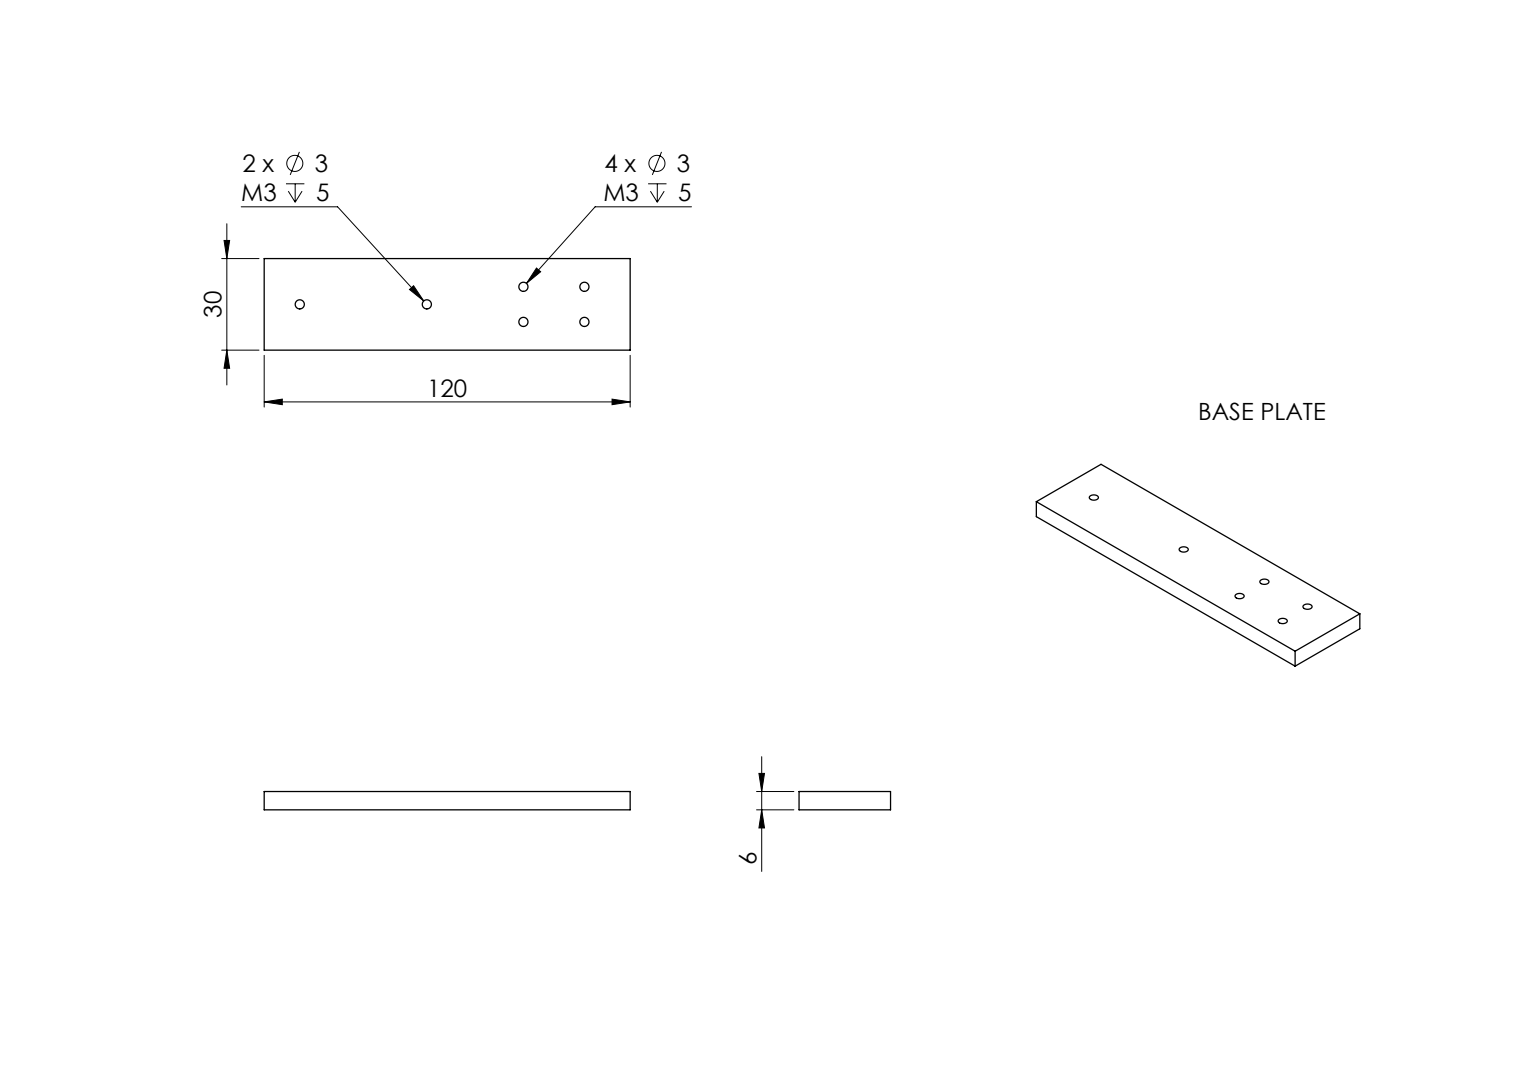
ISO-10303-21;
HEADER;
FILE_DESCRIPTION (('STEP AP214'),
    '1' );
FILE_NAME ('base plate.step',
    '2026-10-26T05:17:54',
    ( '' ),
    ( '' ),
    'SwSTEP 2.0',
    'SolidWorks 2026',
    '' );
FILE_SCHEMA (( 'AUTOMOTIVE_DESIGN' ));
ENDSEC;

DATA;
#8=DIRECTION ( 'NONE',  ( -0.000000000000000000, 1.000000000000000000, -0.000000000000000000 ) ) ;
#20=SURFACE_STYLE_FILL_AREA ( #10773 ) ;
#32=CARTESIAN_POINT ( 'NONE',  ( 45.00000000000000000, 0.000000000000000000, -4.249999999999998224 ) ) ;
#39=VERTEX_POINT ( 'NONE', #7644 ) ;
#40=COLOUR_RGB ( '',0.8941176470588234615, 0.8941176470588234615, 0.8941176470588234615 ) ;
#57=EDGE_CURVE ( 'NONE', #11292, #8351, #9858, .T. ) ;
#75=FACE_BOUND ( 'NONE', #11702, .T. ) ;
#138=DIRECTION ( 'NONE',  ( 0.000000000000000000, 0.000000000000000000, 1.000000000000000000 ) ) ;
#139=DIRECTION ( 'NONE',  ( 0.000000000000000000, -0.000000000000000000, -1.000000000000000000 ) ) ;
#141=ADVANCED_FACE ( 'NONE', ( #3852 ), #10839, .F. ) ;
#168=EDGE_CURVE ( 'NONE', #9993, #9602, #10963, .T. ) ;
#174=EDGE_LOOP ( 'NONE', ( #6858, #8002, #3578, #927 ) ) ;
#212=CARTESIAN_POINT ( 'NONE',  ( -48.33333333333332860, -5.000000000000000000, -1.500000000000003109 ) ) ;
#223=ADVANCED_FACE ( 'NONE', ( #9797 ), #3264, .F. ) ;
#226=DIRECTION ( 'NONE',  ( -0.000000000000000000, 1.000000000000000000, -0.000000000000000000 ) ) ;
#230=ORIENTED_EDGE ( 'NONE', *, *, #426, .T. ) ;
#248=DIRECTION ( 'NONE',  ( 1.049727191973305517E-16, 0.5150380737757253025, -0.8571673013836857979 ) ) ;
#266=LINE ( 'NONE', #12261, #1845 ) ;
#305=ORIENTED_EDGE ( 'NONE', *, *, #8048, .F. ) ;
#309=VERTEX_POINT ( 'NONE', #6189 ) ;
#369=AXIS2_PLACEMENT_3D ( 'NONE', #12355, #9278, #12488 ) ;
#376=VERTEX_POINT ( 'NONE', #8487 ) ;
#382=CARTESIAN_POINT ( 'NONE',  ( 60.00000000000000000, -6.000000000000000000, 15.00000000000000000 ) ) ;
#426=EDGE_CURVE ( 'NONE', #11653, #6806, #2729, .T. ) ;
#432=DIRECTION ( 'NONE',  ( 0.000000000000000000, 0.000000000000000000, 1.000000000000000000 ) ) ;
#469=DIRECTION ( 'NONE',  ( -0.000000000000000000, 1.000000000000000000, -0.000000000000000000 ) ) ;
#487=DIRECTION ( 'NONE',  ( -0.000000000000000000, 1.000000000000000000, -0.000000000000000000 ) ) ;
#502=AXIS2_PLACEMENT_3D ( 'NONE', #7934, #12717, #11921 ) ;
#511=CARTESIAN_POINT ( 'NONE',  ( -6.666666666666660745, 0.000000000000000000, 0.000000000000000000 ) ) ;
#549=VECTOR ( 'NONE', #1621, 1000.000000000000000 ) ;
#554=DIRECTION ( 'NONE',  ( 0.000000000000000000, 0.000000000000000000, 1.000000000000000000 ) ) ;
#561=VECTOR ( 'NONE', #4344, 999.9999999999998863 ) ;
#572=DIRECTION ( 'NONE',  ( -1.000000000000000000, 0.000000000000000000, 0.000000000000000000 ) ) ;
#603=DIRECTION ( 'NONE',  ( 0.000000000000000000, 0.5150380737757253025, 0.8571673013836857979 ) ) ;
#642=ORIENTED_EDGE ( 'NONE', *, *, #5141, .F. ) ;
#646=DIRECTION ( 'NONE',  ( 0.000000000000000000, 0.000000000000000000, 1.000000000000000000 ) ) ;
#661=AXIS2_PLACEMENT_3D ( 'NONE', #10121, #1470, #8480 ) ;
#670=PLANE ( 'NONE',  #6171 ) ;
#691=CARTESIAN_POINT ( 'NONE',  ( 25.00000000000000355, 0.000000000000000000, 4.249999999999998224 ) ) ;
#711=DIRECTION ( 'NONE',  ( 0.000000000000000000, 0.5150380737757253025, 0.8571673013836857979 ) ) ;
#714=AXIS2_PLACEMENT_3D ( 'NONE', #11287, #12341, #11156 ) ;
#718=VERTEX_POINT ( 'NONE', #4225 ) ;
#732=CIRCLE ( 'NONE', #5327, 1.499999999999999556 ) ;
#743=CIRCLE ( 'NONE', #2637, 1.500000000000001332 ) ;
#761=( LENGTH_UNIT ( ) NAMED_UNIT ( * ) SI_UNIT ( .MILLI., .METRE. ) );
#827=CIRCLE ( 'NONE', #4601, 1.500000000000001332 ) ;
#829=ORIENTED_EDGE ( 'NONE', *, *, #3040, .F. ) ;
#834=EDGE_LOOP ( 'NONE', ( #3807, #9213, #11904 ) ) ;
#835=VERTEX_POINT ( 'NONE', #7421 ) ;
#836=CYLINDRICAL_SURFACE ( 'NONE', #9008, 1.500000000000001332 ) ;
#842=ORIENTED_EDGE ( 'NONE', *, *, #4723, .T. ) ;
#873=ADVANCED_FACE ( 'NONE', ( #1662 ), #6562, .F. ) ;
#880=CARTESIAN_POINT ( 'NONE',  ( 60.00000000000000000, 0.000000000000000000, 15.00000000000000000 ) ) ;
#882=( NAMED_UNIT ( * ) SI_UNIT ( $, .STERADIAN. ) SOLID_ANGLE_UNIT ( ) );
#886=CARTESIAN_POINT ( 'NONE',  ( -60.00000000000000000, -6.000000000000000000, 14.99999999999999645 ) ) ;
#921=AXIS2_PLACEMENT_3D ( 'NONE', #2490, #6466, #10462 ) ;
#927=ORIENTED_EDGE ( 'NONE', *, *, #11531, .F. ) ;
#947=SURFACE_SIDE_STYLE ('',( #20 ) ) ;
#961=DIRECTION ( 'NONE',  ( -0.000000000000000000, 1.000000000000000000, -0.000000000000000000 ) ) ;
#964=CARTESIAN_POINT ( 'NONE',  ( 25.00000000000000355, 0.000000000000000000, 5.750000000000000000 ) ) ;
#965=ORIENTED_EDGE ( 'NONE', *, *, #11531, .T. ) ;
#968=ORIENTED_EDGE ( 'NONE', *, *, #12311, .F. ) ;
#991=AXIS2_PLACEMENT_3D ( 'NONE', #6237, #12192, #2261 ) ;
#992=VERTEX_POINT ( 'NONE', #5842 ) ;
#1021=ORIENTED_EDGE ( 'NONE', *, *, #1157, .F. ) ;
#1080=CARTESIAN_POINT ( 'NONE',  ( 45.00000000000000000, -5.000000000000000000, -5.750000000000000000 ) ) ;
#1123=VECTOR ( 'NONE', #2979, 1000.000000000000000 ) ;
#1131=CIRCLE ( 'NONE', #10551, 1.500000000000001332 ) ;
#1145=CARTESIAN_POINT ( 'NONE',  ( 25.00000000000000355, -5.901290925839664858, 5.750000000000000000 ) ) ;
#1149=AXIS2_PLACEMENT_3D ( 'NONE', #11024, #8159, #2079 ) ;
#1150=ORIENTED_EDGE ( 'NONE', *, *, #3390, .T. ) ;
#1157=EDGE_CURVE ( 'NONE', #11476, #11262, #3029, .T. ) ;
#1162=AXIS2_PLACEMENT_3D ( 'NONE', #1080, #9331, #5271 ) ;
#1190=ORIENTED_EDGE ( 'NONE', *, *, #12704, .T. ) ;
#1200=EDGE_CURVE ( 'NONE', #11292, #11250, #10783, .T. ) ;
#1210=VECTOR ( 'NONE', #2174, 1000.000000000000000 ) ;
#1212=ORIENTED_EDGE ( 'NONE', *, *, #4918, .T. ) ;
#1215=FACE_OUTER_BOUND ( 'NONE', #9863, .T. ) ;
#1219=ORIENTED_EDGE ( 'NONE', *, *, #11969, .T. ) ;
#1227=AXIS2_PLACEMENT_3D ( 'NONE', #3244, #11210, #139 ) ;
#1234=ORIENTED_EDGE ( 'NONE', *, *, #11061, .F. ) ;
#1244=ORIENTED_EDGE ( 'NONE', *, *, #5393, .F. ) ;
#1248=AXIS2_PLACEMENT_3D ( 'NONE', #1741, #5729, #4754 ) ;
#1272=EDGE_CURVE ( 'NONE', #9602, #3240, #4770, .T. ) ;
#1314=LINE ( 'NONE', #10350, #3761 ) ;
#1322=ADVANCED_FACE ( 'NONE', ( #5552 ), #9549, .T. ) ;
#1356=DIRECTION ( 'NONE',  ( -0.000000000000000000, 1.000000000000000000, -0.000000000000000000 ) ) ;
#1379=AXIS2_PLACEMENT_3D ( 'NONE', #8945, #961, #3988 ) ;
#1413=VERTEX_POINT ( 'NONE', #1886 ) ;
#1426=VECTOR ( 'NONE', #3530, 999.9999999999998863 ) ;
#1427=VERTEX_POINT ( 'NONE', #4956 ) ;
#1429=ORIENTED_EDGE ( 'NONE', *, *, #5239, .T. ) ;
#1450=DIRECTION ( 'NONE',  ( -0.000000000000000000, 1.000000000000000000, -0.000000000000000000 ) ) ;
#1453=VECTOR ( 'NONE', #6804, 1000.000000000000000 ) ;
#1458=ADVANCED_FACE ( 'NONE', ( #4045 ), #9800, .F. ) ;
#1461=CIRCLE ( 'NONE', #10650, 1.499999999999999556 ) ;
#1463=DIRECTION ( 'NONE',  ( -0.000000000000000000, 1.000000000000000000, -0.000000000000000000 ) ) ;
#1465=FACE_OUTER_BOUND ( 'NONE', #4679, .T. ) ;
#1470=DIRECTION ( 'NONE',  ( -0.000000000000000000, 1.000000000000000000, -0.000000000000000000 ) ) ;
#1475=DIRECTION ( 'NONE',  ( -0.000000000000000000, 1.000000000000000000, -0.000000000000000000 ) ) ;
#1500=CIRCLE ( 'NONE', #661, 1.500000000000001332 ) ;
#1512=ORIENTED_EDGE ( 'NONE', *, *, #4521, .T. ) ;
#1514=EDGE_LOOP ( 'NONE', ( #2019, #3145, #9148, #1219 ) ) ;
#1544=EDGE_CURVE ( 'NONE', #3240, #4006, #11813, .T. ) ;
#1580=AXIS2_PLACEMENT_3D ( 'NONE', #10565, #12391, #2459 ) ;
#1611=CARTESIAN_POINT ( 'NONE',  ( -48.33333333333332860, 0.000000000000000000, 1.499999999999999556 ) ) ;
#1621=DIRECTION ( 'NONE',  ( 1.049727191973305763E-16, 0.5150380737757249694, -0.8571673013836860200 ) ) ;
#1628=CIRCLE ( 'NONE', #6230, 1.500000000000001332 ) ;
#1639=CIRCLE ( 'NONE', #4977, 1.499999999999999556 ) ;
#1660=DIRECTION ( 'NONE',  ( -0.000000000000000000, 1.000000000000000000, -0.000000000000000000 ) ) ;
#1662=FACE_OUTER_BOUND ( 'NONE', #1514, .T. ) ;
#1692=VERTEX_POINT ( 'NONE', #8490 ) ;
#1702=VECTOR ( 'NONE', #1846, 1000.000000000000000 ) ;
#1729=EDGE_CURVE ( 'NONE', #3927, #7180, #732, .T. ) ;
#1741=CARTESIAN_POINT ( 'NONE',  ( 45.00000000000000000, 0.000000000000000000, 5.750000000000000888 ) ) ;
#1762=PRODUCT_DEFINITION_FORMATION_WITH_SPECIFIED_SOURCE ( 'ANY', '', #11480, .NOT_KNOWN. ) ;
#1813=EDGE_CURVE ( 'NONE', #835, #10173, #10698, .T. ) ;
#1836=CARTESIAN_POINT ( 'NONE',  ( 25.00000000000000355, -5.000000000000000000, 4.249999999999998224 ) ) ;
#1837=EDGE_LOOP ( 'NONE', ( #829, #11058 ) ) ;
#1845=VECTOR ( 'NONE', #3309, 999.9999999999998863 ) ;
#1846=DIRECTION ( 'NONE',  ( -0.000000000000000000, 1.000000000000000000, -0.000000000000000000 ) ) ;
#1850=ADVANCED_FACE ( 'NONE', ( #8989 ), #5792, .F. ) ;
#1861=EDGE_CURVE ( 'NONE', #6806, #1692, #2861, .T. ) ;
#1886=CARTESIAN_POINT ( 'NONE',  ( 45.00000000000000000, -5.000000000000000000, -4.249999999999998224 ) ) ;
#1894=VERTEX_POINT ( 'NONE', #8017 ) ;
#1904=AXIS2_PLACEMENT_3D ( 'NONE', #12320, #3368, #6359 ) ;
#1943=ADVANCED_FACE ( 'NONE', ( #7953 ), #12793, .F. ) ;
#1957=EDGE_LOOP ( 'NONE', ( #2157, #3202 ) ) ;
#1966=CARTESIAN_POINT ( 'NONE',  ( 60.00000000000000000, -6.000000000000000000, 15.00000000000000000 ) ) ;
#1967=ORIENTED_EDGE ( 'NONE', *, *, #5239, .F. ) ;
#1990=LINE ( 'NONE', #9109, #3375 ) ;
#2019=ORIENTED_EDGE ( 'NONE', *, *, #7283, .F. ) ;
#2050=CIRCLE ( 'NONE', #4767, 1.500000000000001332 ) ;
#2073=( LENGTH_UNIT ( ) NAMED_UNIT ( * ) SI_UNIT ( .MILLI., .METRE. ) );
#2079=DIRECTION ( 'NONE',  ( 0.000000000000000000, 0.000000000000000000, 1.000000000000000000 ) ) ;
#2096=VERTEX_POINT ( 'NONE', #3116 ) ;
#2102=LINE ( 'NONE', #12040, #7594 ) ;
#2111=ORIENTED_EDGE ( 'NONE', *, *, #9460, .T. ) ;
#2112=VECTOR ( 'NONE', #11928, 1000.000000000000000 ) ;
#2127=EDGE_CURVE ( 'NONE', #718, #309, #8213, .T. ) ;
#2142=DIRECTION ( 'NONE',  ( 0.000000000000000000, 0.000000000000000000, 1.000000000000000000 ) ) ;
#2143=EDGE_CURVE ( 'NONE', #10857, #8362, #12026, .T. ) ;
#2157=ORIENTED_EDGE ( 'NONE', *, *, #5870, .F. ) ;
#2167=ORIENTED_EDGE ( 'NONE', *, *, #4353, .T. ) ;
#2174=DIRECTION ( 'NONE',  ( 0.000000000000000000, 0.000000000000000000, -1.000000000000000000 ) ) ;
#2201=ADVANCED_FACE ( 'NONE', ( #1465 ), #670, .T. ) ;
#2249=ORIENTED_EDGE ( 'NONE', *, *, #57, .T. ) ;
#2250=EDGE_CURVE ( 'NONE', #2096, #9602, #2849, .T. ) ;
#2261=DIRECTION ( 'NONE',  ( 0.000000000000000000, 0.000000000000000000, 1.000000000000000000 ) ) ;
#2262=PLANE ( 'NONE',  #1227 ) ;
#2292=PLANE ( 'NONE',  #369 ) ;
#2299=EDGE_CURVE ( 'NONE', #4333, #3861, #12859, .T. ) ;
#2307=LINE ( 'NONE', #8254, #11740 ) ;
#2326=CARTESIAN_POINT ( 'NONE',  ( 25.00000000000000355, 0.000000000000000000, 7.250000000000000888 ) ) ;
#2376=ORIENTED_EDGE ( 'NONE', *, *, #5336, .F. ) ;
#2431=DIRECTION ( 'NONE',  ( 0.000000000000000000, 0.000000000000000000, 1.000000000000000000 ) ) ;
#2451=DIRECTION ( 'NONE',  ( -0.000000000000000000, 1.000000000000000000, -0.000000000000000000 ) ) ;
#2459=DIRECTION ( 'NONE',  ( 0.000000000000000000, 0.000000000000000000, 1.000000000000000000 ) ) ;
#2463=DIRECTION ( 'NONE',  ( -0.000000000000000000, 1.000000000000000000, -0.000000000000000000 ) ) ;
#2470=CARTESIAN_POINT ( 'NONE',  ( 25.00000000000000355, -5.000000000000000000, -4.249999999999998224 ) ) ;
#2480=ORIENTED_EDGE ( 'NONE', *, *, #8048, .T. ) ;
#2490=CARTESIAN_POINT ( 'NONE',  ( 45.00000000000000000, 0.000000000000000000, -5.750000000000000000 ) ) ;
#2515=APPLICATION_CONTEXT ( 'automotive_design' ) ;
#2522=CARTESIAN_POINT ( 'NONE',  ( -48.33333333333332860, 0.000000000000000000, -1.734723475976807094E-15 ) ) ;
#2523=DIRECTION ( 'NONE',  ( 0.000000000000000000, -0.000000000000000000, -1.000000000000000000 ) ) ;
#2528=AXIS2_PLACEMENT_3D ( 'NONE', #6434, #12203, #4480 ) ;
#2585=DIRECTION ( 'NONE',  ( -0.000000000000000000, 1.000000000000000000, -0.000000000000000000 ) ) ;
#2600=FACE_OUTER_BOUND ( 'NONE', #10043, .T. ) ;
#2636=EDGE_CURVE ( 'NONE', #6649, #7180, #12447, .T. ) ;
#2637=AXIS2_PLACEMENT_3D ( 'NONE', #9130, #12147, #10308 ) ;
#2658=ORIENTED_EDGE ( 'NONE', *, *, #1813, .T. ) ;
#2697=EDGE_CURVE ( 'NONE', #8362, #12765, #2102, .T. ) ;
#2729=LINE ( 'NONE', #2470, #11141 ) ;
#2730=DIRECTION ( 'NONE',  ( -1.000000000000000000, -0.000000000000000000, -0.000000000000000000 ) ) ;
#2740=FACE_OUTER_BOUND ( 'NONE', #11021, .T. ) ;
#2763=APPLICATION_CONTEXT ( 'automotive_design' ) ;
#2809=ORIENTED_EDGE ( 'NONE', *, *, #5336, .T. ) ;
#2825=ORIENTED_EDGE ( 'NONE', *, *, #3804, .F. ) ;
#2849=CIRCLE ( 'NONE', #10145, 1.500000000000001332 ) ;
#2861=LINE ( 'NONE', #5855, #8272 ) ;
#2868=CIRCLE ( 'NONE', #6403, 1.500000000000001332 ) ;
#2884=EDGE_LOOP ( 'NONE', ( #11242, #3591, #10722 ) ) ;
#2902=FACE_OUTER_BOUND ( 'NONE', #7339, .T. ) ;
#2922=DIRECTION ( 'NONE',  ( -0.000000000000000000, 1.000000000000000000, -0.000000000000000000 ) ) ;
#2941=LINE ( 'NONE', #32, #8499 ) ;
#2956=ORIENTED_EDGE ( 'NONE', *, *, #9180, .F. ) ;
#2970=VERTEX_POINT ( 'NONE', #1145 ) ;
#2979=DIRECTION ( 'NONE',  ( -0.000000000000000000, -0.000000000000000000, 1.000000000000000000 ) ) ;
#3018=CARTESIAN_POINT ( 'NONE',  ( 45.00000000000000000, 0.000000000000000000, -7.250000000000000888 ) ) ;
#3021=CIRCLE ( 'NONE', #5091, 1.500000000000001332 ) ;
#3029=CIRCLE ( 'NONE', #921, 1.500000000000001332 ) ;
#3040=EDGE_CURVE ( 'NONE', #4006, #3240, #743, .T. ) ;
#3041=ADVANCED_FACE ( 'NONE', ( #1215 ), #8221, .F. ) ;
#3048=EDGE_CURVE ( 'NONE', #1413, #39, #9521, .T. ) ;
#3063=CARTESIAN_POINT ( 'NONE',  ( 25.00000000000000355, 0.000000000000000000, -5.750000000000000000 ) ) ;
#3088=ORIENTED_EDGE ( 'NONE', *, *, #9280, .F. ) ;
#3110=DIRECTION ( 'NONE',  ( -0.000000000000000000, 1.000000000000000000, -0.000000000000000000 ) ) ;
#3113=CIRCLE ( 'NONE', #3943, 1.500000000000001332 ) ;
#3116=CARTESIAN_POINT ( 'NONE',  ( 45.00000000000000000, -5.000000000000000000, 7.250000000000001776 ) ) ;
#3117=AXIS2_PLACEMENT_3D ( 'NONE', #3412, #3288, #2431 ) ;
#3140=EDGE_LOOP ( 'NONE', ( #3540, #7051, #10160 ) ) ;
#3145=ORIENTED_EDGE ( 'NONE', *, *, #2299, .F. ) ;
#3171=ORIENTED_EDGE ( 'NONE', *, *, #4593, .F. ) ;
#3199=ORIENTED_EDGE ( 'NONE', *, *, #1813, .F. ) ;
#3202=ORIENTED_EDGE ( 'NONE', *, *, #10109, .F. ) ;
#3229=ORIENTED_EDGE ( 'NONE', *, *, #4593, .T. ) ;
#3240=VERTEX_POINT ( 'NONE', #7653 ) ;
#3244=CARTESIAN_POINT ( 'NONE',  ( 0.000000000000000000, 0.000000000000000000, 0.000000000000000000 ) ) ;
#3250=DIRECTION ( 'NONE',  ( 0.000000000000000000, 0.5150380737757255245, 0.8571673013836856869 ) ) ;
#3263=AXIS2_PLACEMENT_3D ( 'NONE', #4676, #7551, #8541 ) ;
#3264=CYLINDRICAL_SURFACE ( 'NONE', #9272, 1.500000000000001332 ) ;
#3288=DIRECTION ( 'NONE',  ( -0.000000000000000000, 1.000000000000000000, -0.000000000000000000 ) ) ;
#3289=ORIENTED_EDGE ( 'NONE', *, *, #8865, .F. ) ;
#3309=DIRECTION ( 'NONE',  ( 1.049727191973305517E-16, 0.5150380737757253025, -0.8571673013836857979 ) ) ;
#3310=FACE_BOUND ( 'NONE', #1957, .T. ) ;
#3316=FACE_OUTER_BOUND ( 'NONE', #7620, .T. ) ;
#3322=ORIENTED_EDGE ( 'NONE', *, *, #2636, .F. ) ;
#3328=EDGE_CURVE ( 'NONE', #1894, #4333, #10846, .T. ) ;
#3362=ADVANCED_FACE ( 'NONE', ( #9995 ), #9730, .F. ) ;
#3368=DIRECTION ( 'NONE',  ( -0.000000000000000000, 1.000000000000000000, -0.000000000000000000 ) ) ;
#3375=VECTOR ( 'NONE', #4085, 1000.000000000000000 ) ;
#3383=EDGE_LOOP ( 'NONE', ( #1967, #230, #5298 ) ) ;
#3390=EDGE_CURVE ( 'NONE', #1413, #11262, #2941, .T. ) ;
#3412=CARTESIAN_POINT ( 'NONE',  ( 25.00000000000000355, -5.000000000000000000, 5.750000000000000000 ) ) ;
#3413=EDGE_LOOP ( 'NONE', ( #12358, #9333, #11344, #12552 ) ) ;
#3464=ORIENTED_EDGE ( 'NONE', *, *, #9180, .T. ) ;
#3468=FACE_OUTER_BOUND ( 'NONE', #3902, .T. ) ;
#3481=ORIENTED_EDGE ( 'NONE', *, *, #426, .F. ) ;
#3485=UNCERTAINTY_MEASURE_WITH_UNIT (LENGTH_MEASURE( 1.000000000000000082E-05 ), #761, 'distance_accuracy_value', 'NONE');
#3506=AXIS2_PLACEMENT_3D ( 'NONE', #11285, #4103, #10303 ) ;
#3530=DIRECTION ( 'NONE',  ( 0.000000000000000000, 0.5150380737757253025, 0.8571673013836857979 ) ) ;
#3540=ORIENTED_EDGE ( 'NONE', *, *, #12418, .F. ) ;
#3546=DIRECTION ( 'NONE',  ( 0.000000000000000000, 0.000000000000000000, -1.000000000000000000 ) ) ;
#3570=FACE_OUTER_BOUND ( 'NONE', #10154, .T. ) ;
#3578=ORIENTED_EDGE ( 'NONE', *, *, #1544, .T. ) ;
#3581=LINE ( 'NONE', #1611, #6563 ) ;
#3591=ORIENTED_EDGE ( 'NONE', *, *, #2127, .T. ) ;
#3611=ORIENTED_EDGE ( 'NONE', *, *, #9460, .F. ) ;
#3624=VECTOR ( 'NONE', #711, 999.9999999999998863 ) ;
#3631=( GEOMETRIC_REPRESENTATION_CONTEXT ( 3 ) GLOBAL_UNCERTAINTY_ASSIGNED_CONTEXT ( ( #12637 ) ) GLOBAL_UNIT_ASSIGNED_CONTEXT ( ( #2073, #8874, #882 ) ) REPRESENTATION_CONTEXT ( 'NONE', 'WORKASPACE' ) );
#3701=CARTESIAN_POINT ( 'NONE',  ( 0.000000000000000000, -6.000000000000000000, 0.000000000000000000 ) ) ;
#3710=DIRECTION ( 'NONE',  ( 0.000000000000000000, 0.5150380737757253025, 0.8571673013836857979 ) ) ;
#3726=AXIS2_PLACEMENT_3D ( 'NONE', #8336, #8271, #138 ) ;
#3739=LINE ( 'NONE', #12757, #3624 ) ;
#3761=VECTOR ( 'NONE', #9303, 1000.000000000000000 ) ;
#3782=CARTESIAN_POINT ( 'NONE',  ( -60.00000000000000000, 0.000000000000000000, 14.99999999999999645 ) ) ;
#3784=FACE_BOUND ( 'NONE', #4596, .T. ) ;
#3790=LINE ( 'NONE', #7769, #11042 ) ;
#3804=EDGE_CURVE ( 'NONE', #1692, #7167, #2868, .T. ) ;
#3807=ORIENTED_EDGE ( 'NONE', *, *, #4521, .F. ) ;
#3847=( NAMED_UNIT ( * ) PLANE_ANGLE_UNIT ( ) SI_UNIT ( $, .RADIAN. ) );
#3852=FACE_OUTER_BOUND ( 'NONE', #3413, .T. ) ;
#3860=AXIS2_PLACEMENT_3D ( 'NONE', #12668, #1475, #4688 ) ;
#3861=VERTEX_POINT ( 'NONE', #212 ) ;
#3897=LINE ( 'NONE', #4932, #2112 ) ;
#3902=EDGE_LOOP ( 'NONE', ( #3289, #9942, #2249, #1190 ) ) ;
#3927=VERTEX_POINT ( 'NONE', #5387 ) ;
#3934=AXIS2_PLACEMENT_3D ( 'NONE', #7413, #6423, #9506 ) ;
#3943=AXIS2_PLACEMENT_3D ( 'NONE', #5939, #9938, #6203 ) ;
#3986=ORIENTED_EDGE ( 'NONE', *, *, #1729, .F. ) ;
#3988=DIRECTION ( 'NONE',  ( 0.000000000000000000, 0.000000000000000000, 1.000000000000000000 ) ) ;
#4006=VERTEX_POINT ( 'NONE', #6435 ) ;
#4039=PRESENTATION_STYLE_ASSIGNMENT (( #6052 ) ) ;
#4045=FACE_OUTER_BOUND ( 'NONE', #7966, .T. ) ;
#4049=DIRECTION ( 'NONE',  ( 0.000000000000000000, 0.5150380737757249694, 0.8571673013836860200 ) ) ;
#4058=ORIENTED_EDGE ( 'NONE', *, *, #7681, .F. ) ;
#4082=CONICAL_SURFACE ( 'NONE', #502, 1.500000000000001332, 1.029744260000000411 ) ;
#4085=DIRECTION ( 'NONE',  ( 0.000000000000000000, 1.000000000000000000, 0.000000000000000000 ) ) ;
#4089=DIRECTION ( 'NONE',  ( 0.000000000000000000, 0.000000000000000000, 1.000000000000000000 ) ) ;
#4103=DIRECTION ( 'NONE',  ( -0.000000000000000000, 1.000000000000000000, -0.000000000000000000 ) ) ;
#4135=DIRECTION ( 'NONE',  ( 0.000000000000000000, 0.000000000000000000, -1.000000000000000000 ) ) ;
#4206=CONICAL_SURFACE ( 'NONE', #11920, 1.500000000000001332, 1.029744260000000411 ) ;
#4215=PRODUCT_DEFINITION_CONTEXT ( 'detailed design', #2763, 'design' ) ;
#4225=CARTESIAN_POINT ( 'NONE',  ( -6.666666666666660745, -5.901290925839663970, 0.000000000000000000 ) ) ;
#4249=LINE ( 'NONE', #8171, #5695 ) ;
#4253=STYLED_ITEM ( 'NONE', ( #4039 ), #11356 ) ;
#4257=VECTOR ( 'NONE', #1450, 1000.000000000000000 ) ;
#4283=CARTESIAN_POINT ( 'NONE',  ( 25.00000000000000355, -5.000000000000000000, 4.249999999999998224 ) ) ;
#4286=EDGE_CURVE ( 'NONE', #8362, #10857, #11427, .T. ) ;
#4306=DIRECTION ( 'NONE',  ( -0.000000000000000000, 1.000000000000000000, -0.000000000000000000 ) ) ;
#4333=VERTEX_POINT ( 'NONE', #5041 ) ;
#4344=DIRECTION ( 'NONE',  ( 1.049727191973305517E-16, 0.5150380737757253025, -0.8571673013836857979 ) ) ;
#4353=EDGE_CURVE ( 'NONE', #4553, #835, #5953, .T. ) ;
#4390=ADVANCED_FACE ( 'NONE', ( #12678 ), #7671, .F. ) ;
#4417=DIRECTION ( 'NONE',  ( 0.000000000000000000, 0.000000000000000000, 1.000000000000000000 ) ) ;
#4427=FACE_OUTER_BOUND ( 'NONE', #2884, .T. ) ;
#4440=DIRECTION ( 'NONE',  ( -0.000000000000000000, 1.000000000000000000, -0.000000000000000000 ) ) ;
#4465=ORIENTED_EDGE ( 'NONE', *, *, #5254, .T. ) ;
#4480=DIRECTION ( 'NONE',  ( 0.000000000000000000, 0.000000000000000000, 1.000000000000000000 ) ) ;
#4521=EDGE_CURVE ( 'NONE', #1894, #3861, #5733, .T. ) ;
#4532=CARTESIAN_POINT ( 'NONE',  ( -6.666666666666660745, 0.000000000000000000, -1.499999999999999556 ) ) ;
#4545=AXIS2_PLACEMENT_3D ( 'NONE', #5770, #8838, #9634 ) ;
#4553=VERTEX_POINT ( 'NONE', #880 ) ;
#4572=CARTESIAN_POINT ( 'NONE',  ( 45.00000000000000000, -5.000000000000000000, 7.250000000000001776 ) ) ;
#4575=CARTESIAN_POINT ( 'NONE',  ( -6.666666666666660745, 0.000000000000000000, -1.499999999999999556 ) ) ;
#4579=DIRECTION ( 'NONE',  ( 0.000000000000000000, 0.000000000000000000, 1.000000000000000000 ) ) ;
#4593=EDGE_CURVE ( 'NONE', #10173, #11250, #8933, .T. ) ;
#4596=EDGE_LOOP ( 'NONE', ( #5931, #9274 ) ) ;
#4601=AXIS2_PLACEMENT_3D ( 'NONE', #7047, #9004, #5213 ) ;
#4604=( NAMED_UNIT ( * ) PLANE_ANGLE_UNIT ( ) SI_UNIT ( $, .RADIAN. ) );
#4629=ORIENTED_EDGE ( 'NONE', *, *, #3390, .F. ) ;
#4632=EDGE_LOOP ( 'NONE', ( #305, #8686, #7211, #4629 ) ) ;
#4633=DIRECTION ( 'NONE',  ( 0.000000000000000000, 0.000000000000000000, 1.000000000000000000 ) ) ;
#4653=PLANE ( 'NONE',  #11336 ) ;
#4676=CARTESIAN_POINT ( 'NONE',  ( 25.00000000000000355, -5.000000000000000000, 5.750000000000000000 ) ) ;
#4679=EDGE_LOOP ( 'NONE', ( #1244, #11959, #7907, #3611 ) ) ;
#4688=DIRECTION ( 'NONE',  ( 0.000000000000000000, 0.000000000000000000, 1.000000000000000000 ) ) ;
#4708=DIRECTION ( 'NONE',  ( -0.000000000000000000, 1.000000000000000000, -0.000000000000000000 ) ) ;
#4722=VECTOR ( 'NONE', #3250, 999.9999999999998863 ) ;
#4723=EDGE_CURVE ( 'NONE', #1427, #992, #9128, .T. ) ;
#4742=EDGE_CURVE ( 'NONE', #718, #6649, #11085, .T. ) ;
#4754=DIRECTION ( 'NONE',  ( 0.000000000000000000, 0.000000000000000000, 1.000000000000000000 ) ) ;
#4767=AXIS2_PLACEMENT_3D ( 'NONE', #9572, #2451, #6555 ) ;
#4770=LINE ( 'NONE', #6658, #12645 ) ;
#4824=DIRECTION ( 'NONE',  ( 0.000000000000000000, 0.000000000000000000, 1.000000000000000000 ) ) ;
#4825=FACE_BOUND ( 'NONE', #1837, .T. ) ;
#4874=CARTESIAN_POINT ( 'NONE',  ( -60.00000000000000000, -6.000000000000000000, 14.99999999999999645 ) ) ;
#4886=DIRECTION ( 'NONE',  ( 1.000000000000000000, 0.000000000000000000, 0.000000000000000000 ) ) ;
#4894=CARTESIAN_POINT ( 'NONE',  ( -6.666666666666660745, 0.000000000000000000, 0.000000000000000000 ) ) ;
#4918=EDGE_CURVE ( 'NONE', #10857, #6375, #7622, .T. ) ;
#4932=CARTESIAN_POINT ( 'NONE',  ( 45.00000000000000000, 0.000000000000000000, -7.250000000000000888 ) ) ;
#4956=CARTESIAN_POINT ( 'NONE',  ( -48.33333333333332860, 0.000000000000000000, -1.500000000000003109 ) ) ;
#4959=EDGE_LOOP ( 'NONE', ( #3986, #7360 ) ) ;
#4970=EDGE_LOOP ( 'NONE', ( #10182, #7587, #1212, #10396 ) ) ;
#4977=AXIS2_PLACEMENT_3D ( 'NONE', #11301, #1356, #432 ) ;
#5029=ORIENTED_EDGE ( 'NONE', *, *, #5954, .T. ) ;
#5030=ORIENTED_EDGE ( 'NONE', *, *, #9280, .T. ) ;
#5041=CARTESIAN_POINT ( 'NONE',  ( -48.33333333333332860, -5.000000000000000000, 1.499999999999999556 ) ) ;
#5051=( GEOMETRIC_REPRESENTATION_CONTEXT ( 3 ) GLOBAL_UNCERTAINTY_ASSIGNED_CONTEXT ( ( #11450 ) ) GLOBAL_UNIT_ASSIGNED_CONTEXT ( ( #11723, #4604, #8717 ) ) REPRESENTATION_CONTEXT ( 'NONE', 'WORKASPACE' ) );
#5059=AXIS2_PLACEMENT_3D ( 'NONE', #6650, #4440, #5612 ) ;
#5068=CARTESIAN_POINT ( 'NONE',  ( -6.666666666666660745, -5.000000000000000000, -1.499999999999999556 ) ) ;
#5091=AXIS2_PLACEMENT_3D ( 'NONE', #7752, #8, #10825 ) ;
#5114=VECTOR ( 'NONE', #11306, 1000.000000000000000 ) ;
#5118=EDGE_CURVE ( 'NONE', #6806, #376, #6219, .T. ) ;
#5131=EDGE_CURVE ( 'NONE', #2970, #8362, #7286, .T. ) ;
#5141=EDGE_CURVE ( 'NONE', #3861, #4333, #7884, .T. ) ;
#5157=ORIENTED_EDGE ( 'NONE', *, *, #1272, .F. ) ;
#5172=LINE ( 'NONE', #8061, #1210 ) ;
#5201=EDGE_LOOP ( 'NONE', ( #3199, #7911, #2111, #10283 ) ) ;
#5202=EDGE_CURVE ( 'NONE', #11262, #11476, #7482, .T. ) ;
#5213=DIRECTION ( 'NONE',  ( 0.000000000000000000, 0.000000000000000000, 1.000000000000000000 ) ) ;
#5239=EDGE_CURVE ( 'NONE', #11653, #376, #266, .T. ) ;
#5254=EDGE_CURVE ( 'NONE', #6459, #835, #10422, .T. ) ;
#5271=DIRECTION ( 'NONE',  ( 0.000000000000000000, 0.000000000000000000, 1.000000000000000000 ) ) ;
#5296=ADVANCED_FACE ( 'NONE', ( #7543 ), #11230, .F. ) ;
#5298=ORIENTED_EDGE ( 'NONE', *, *, #5118, .T. ) ;
#5327=AXIS2_PLACEMENT_3D ( 'NONE', #7566, #5534, #554 ) ;
#5329=EDGE_LOOP ( 'NONE', ( #8349, #9058, #5030 ) ) ;
#5336=EDGE_CURVE ( 'NONE', #7167, #1692, #2050, .T. ) ;
#5387=CARTESIAN_POINT ( 'NONE',  ( -6.666666666666660745, 0.000000000000000000, 1.499999999999999556 ) ) ;
#5393=EDGE_CURVE ( 'NONE', #8351, #6459, #5172, .T. ) ;
#5436=EDGE_CURVE ( 'NONE', #9602, #2096, #1628, .T. ) ;
#5438=AXIS2_PLACEMENT_3D ( 'NONE', #8661, #1463, #7613 ) ;
#5447=CARTESIAN_POINT ( 'NONE',  ( 25.00000000000000355, -5.000000000000000000, -4.249999999999998224 ) ) ;
#5492=MECHANICAL_DESIGN_GEOMETRIC_PRESENTATION_REPRESENTATION('',(#4253),#5909);
#5498=ORIENTED_EDGE ( 'NONE', *, *, #9982, .T. ) ;
#5503=SHAPE_REPRESENTATION ( 'base plate', ( #5704 ), #3631 ) ;
#5513=ADVANCED_FACE ( 'NONE', ( #6605 ), #9488, .T. ) ;
#5534=DIRECTION ( 'NONE',  ( -0.000000000000000000, 1.000000000000000000, -0.000000000000000000 ) ) ;
#5552=FACE_OUTER_BOUND ( 'NONE', #11713, .T. ) ;
#5553=SHAPE_DEFINITION_REPRESENTATION ( #7516, #5503 ) ;
#5612=DIRECTION ( 'NONE',  ( 0.000000000000000000, 0.000000000000000000, 1.000000000000000000 ) ) ;
#5632=AXIS2_PLACEMENT_3D ( 'NONE', #12838, #10867, #9887 ) ;
#5695=VECTOR ( 'NONE', #6202, 1000.000000000000000 ) ;
#5700=CARTESIAN_POINT ( 'NONE',  ( 25.00000000000000355, 0.000000000000000000, -7.250000000000000888 ) ) ;
#5704=AXIS2_PLACEMENT_3D ( 'NONE', #8997, #4824, #4886 ) ;
#5711=FACE_OUTER_BOUND ( 'NONE', #3140, .T. ) ;
#5722=ORIENTED_EDGE ( 'NONE', *, *, #2636, .T. ) ;
#5729=DIRECTION ( 'NONE',  ( -0.000000000000000000, 1.000000000000000000, -0.000000000000000000 ) ) ;
#5733=LINE ( 'NONE', #6584, #549 ) ;
#5770=CARTESIAN_POINT ( 'NONE',  ( 25.00000000000000355, -5.000000000000000000, 5.750000000000000000 ) ) ;
#5792=CYLINDRICAL_SURFACE ( 'NONE', #10971, 1.500000000000001332 ) ;
#5826=CONICAL_SURFACE ( 'NONE', #3117, 1.500000000000001332, 1.029744260000000411 ) ;
#5830=LINE ( 'NONE', #6809, #1702 ) ;
#5833=VECTOR ( 'NONE', #603, 999.9999999999998863 ) ;
#5842=CARTESIAN_POINT ( 'NONE',  ( -48.33333333333332860, 0.000000000000000000, 1.499999999999999556 ) ) ;
#5851=AXIS2_PLACEMENT_3D ( 'NONE', #7309, #487, #11489 ) ;
#5855=CARTESIAN_POINT ( 'NONE',  ( 25.00000000000000355, 0.000000000000000000, -4.249999999999998224 ) ) ;
#5870=EDGE_CURVE ( 'NONE', #6375, #12765, #3113, .T. ) ;
#5891=MECHANICAL_DESIGN_GEOMETRIC_PRESENTATION_REPRESENTATION('',(#8407),#5051);
#5909=( GEOMETRIC_REPRESENTATION_CONTEXT ( 3 ) GLOBAL_UNCERTAINTY_ASSIGNED_CONTEXT ( ( #3485 ) ) GLOBAL_UNIT_ASSIGNED_CONTEXT ( ( #761, #3847, #6844 ) ) REPRESENTATION_CONTEXT ( 'NONE', 'WORKASPACE' ) );
#5921=EDGE_CURVE ( 'NONE', #309, #6649, #1639, .T. ) ;
#5931=ORIENTED_EDGE ( 'NONE', *, *, #11969, .F. ) ;
#5939=CARTESIAN_POINT ( 'NONE',  ( 25.00000000000000355, 0.000000000000000000, 5.750000000000000000 ) ) ;
#5948=VECTOR ( 'NONE', #2730, 1000.000000000000000 ) ;
#5953=LINE ( 'NONE', #9950, #9551 ) ;
#5954=EDGE_CURVE ( 'NONE', #9993, #2096, #6393, .T. ) ;
#5980=DIRECTION ( 'NONE',  ( 0.000000000000000000, 0.000000000000000000, 1.000000000000000000 ) ) ;
#5992=ADVANCED_FACE ( 'NONE', ( #3468 ), #2292, .T. ) ;
#6045=CARTESIAN_POINT ( 'NONE',  ( 45.00000000000000000, 0.000000000000000000, 5.750000000000000888 ) ) ;
#6052=SURFACE_STYLE_USAGE ( .BOTH. , #947 ) ;
#6079=EDGE_LOOP ( 'NONE', ( #2956, #10660, #2480 ) ) ;
#6171=AXIS2_PLACEMENT_3D ( 'NONE', #3701, #8664, #2523 ) ;
#6189=CARTESIAN_POINT ( 'NONE',  ( -6.666666666666660745, -5.000000000000000000, 1.499999999999999556 ) ) ;
#6202=DIRECTION ( 'NONE',  ( 0.000000000000000000, 1.000000000000000000, 0.000000000000000000 ) ) ;
#6203=DIRECTION ( 'NONE',  ( 0.000000000000000000, 0.000000000000000000, 1.000000000000000000 ) ) ;
#6207=AXIS2_PLACEMENT_3D ( 'NONE', #10585, #10644, #4633 ) ;
#6219=CIRCLE ( 'NONE', #7892, 1.500000000000001332 ) ;
#6230=AXIS2_PLACEMENT_3D ( 'NONE', #9098, #7206, #7332 ) ;
#6233=ORIENTED_EDGE ( 'NONE', *, *, #5131, .F. ) ;
#6237=CARTESIAN_POINT ( 'NONE',  ( 45.00000000000000000, 0.000000000000000000, -5.750000000000000000 ) ) ;
#6240=ADVANCED_FACE ( 'NONE', ( #3784, #10774, #4825, #3310, #8079, #75, #12325 ), #2262, .F. ) ;
#6320=CYLINDRICAL_SURFACE ( 'NONE', #5851, 1.500000000000001332 ) ;
#6359=DIRECTION ( 'NONE',  ( 0.000000000000000000, 0.000000000000000000, 1.000000000000000000 ) ) ;
#6375=VERTEX_POINT ( 'NONE', #2326 ) ;
#6377=DIRECTION ( 'NONE',  ( 1.049727191973305394E-16, 0.5150380737757255245, -0.8571673013836856869 ) ) ;
#6378=ORIENTED_EDGE ( 'NONE', *, *, #1729, .T. ) ;
#6393=LINE ( 'NONE', #4572, #1426 ) ;
#6403=AXIS2_PLACEMENT_3D ( 'NONE', #12271, #8086, #12204 ) ;
#6423=DIRECTION ( 'NONE',  ( -0.000000000000000000, 1.000000000000000000, -0.000000000000000000 ) ) ;
#6434=CARTESIAN_POINT ( 'NONE',  ( -48.33333333333332860, 0.000000000000000000, -1.734723475976807094E-15 ) ) ;
#6435=CARTESIAN_POINT ( 'NONE',  ( 45.00000000000000000, 0.000000000000000000, 7.250000000000001776 ) ) ;
#6459=VERTEX_POINT ( 'NONE', #9439 ) ;
#6462=ORIENTED_EDGE ( 'NONE', *, *, #3040, .T. ) ;
#6466=DIRECTION ( 'NONE',  ( -0.000000000000000000, 1.000000000000000000, -0.000000000000000000 ) ) ;
#6555=DIRECTION ( 'NONE',  ( 0.000000000000000000, 0.000000000000000000, 1.000000000000000000 ) ) ;
#6559=ADVANCED_FACE ( 'NONE', ( #12104 ), #5826, .F. ) ;
#6562=CYLINDRICAL_SURFACE ( 'NONE', #8861, 1.500000000000001332 ) ;
#6563=VECTOR ( 'NONE', #9589, 1000.000000000000000 ) ;
#6572=FACE_OUTER_BOUND ( 'NONE', #834, .T. ) ;
#6584=CARTESIAN_POINT ( 'NONE',  ( -48.33333333333332860, -5.000000000000000000, -1.500000000000003109 ) ) ;
#6605=FACE_OUTER_BOUND ( 'NONE', #8112, .T. ) ;
#6627=DIRECTION ( 'NONE',  ( -0.000000000000000000, 1.000000000000000000, -0.000000000000000000 ) ) ;
#6649=VERTEX_POINT ( 'NONE', #9441 ) ;
#6650=CARTESIAN_POINT ( 'NONE',  ( 45.00000000000000000, -5.000000000000000000, 5.750000000000000888 ) ) ;
#6658=CARTESIAN_POINT ( 'NONE',  ( 45.00000000000000000, 0.000000000000000000, 4.249999999999999112 ) ) ;
#6667=DIRECTION ( 'NONE',  ( -0.000000000000000000, 1.000000000000000000, -0.000000000000000000 ) ) ;
#6690=LINE ( 'NONE', #8723, #5833 ) ;
#6708=CYLINDRICAL_SURFACE ( 'NONE', #1248, 1.500000000000001332 ) ;
#6804=DIRECTION ( 'NONE',  ( -0.000000000000000000, 1.000000000000000000, -0.000000000000000000 ) ) ;
#6806=VERTEX_POINT ( 'NONE', #5447 ) ;
#6809=CARTESIAN_POINT ( 'NONE',  ( 45.00000000000000000, 0.000000000000000000, 7.250000000000001776 ) ) ;
#6830=VECTOR ( 'NONE', #6377, 999.9999999999998863 ) ;
#6839=VERTEX_POINT ( 'NONE', #11726 ) ;
#6844=( NAMED_UNIT ( * ) SI_UNIT ( $, .STERADIAN. ) SOLID_ANGLE_UNIT ( ) );
#6858=ORIENTED_EDGE ( 'NONE', *, *, #5436, .F. ) ;
#6866=EDGE_LOOP ( 'NONE', ( #6233, #7189, #9486 ) ) ;
#6918=ADVANCED_FACE ( 'NONE', ( #2902 ), #8764, .F. ) ;
#6953=ORIENTED_EDGE ( 'NONE', *, *, #10948, .F. ) ;
#6968=ORIENTED_EDGE ( 'NONE', *, *, #2697, .T. ) ;
#6970=ORIENTED_EDGE ( 'NONE', *, *, #5393, .T. ) ;
#7000=LINE ( 'NONE', #5700, #1453 ) ;
#7047=CARTESIAN_POINT ( 'NONE',  ( 25.00000000000000355, 0.000000000000000000, 5.750000000000000000 ) ) ;
#7051=ORIENTED_EDGE ( 'NONE', *, *, #5131, .T. ) ;
#7114=ORIENTED_EDGE ( 'NONE', *, *, #8598, .T. ) ;
#7167=VERTEX_POINT ( 'NONE', #8749 ) ;
#7175=CARTESIAN_POINT ( 'NONE',  ( 45.00000000000000000, -5.901290925839664858, 5.750000000000000888 ) ) ;
#7180=VERTEX_POINT ( 'NONE', #4575 ) ;
#7189=ORIENTED_EDGE ( 'NONE', *, *, #12418, .T. ) ;
#7206=DIRECTION ( 'NONE',  ( -0.000000000000000000, 1.000000000000000000, -0.000000000000000000 ) ) ;
#7211=ORIENTED_EDGE ( 'NONE', *, *, #1157, .T. ) ;
#7236=ORIENTED_EDGE ( 'NONE', *, *, #9746, .T. ) ;
#7243=DIRECTION ( 'NONE',  ( -0.000000000000000000, 1.000000000000000000, -0.000000000000000000 ) ) ;
#7283=EDGE_CURVE ( 'NONE', #3861, #1427, #10837, .T. ) ;
#7286=LINE ( 'NONE', #4283, #561 ) ;
#7301=AXIS2_PLACEMENT_3D ( 'NONE', #10811, #8912, #12907 ) ;
#7309=CARTESIAN_POINT ( 'NONE',  ( 25.00000000000000355, 0.000000000000000000, -5.750000000000000000 ) ) ;
#7332=DIRECTION ( 'NONE',  ( 0.000000000000000000, 0.000000000000000000, 1.000000000000000000 ) ) ;
#7339=EDGE_LOOP ( 'NONE', ( #12515, #1512, #10815 ) ) ;
#7345=CARTESIAN_POINT ( 'NONE',  ( 45.00000000000000000, 0.000000000000000000, -4.249999999999998224 ) ) ;
#7360=ORIENTED_EDGE ( 'NONE', *, *, #9982, .F. ) ;
#7371=CARTESIAN_POINT ( 'NONE',  ( -60.00000000000000000, 0.000000000000000000, -15.00000000000000355 ) ) ;
#7413=CARTESIAN_POINT ( 'NONE',  ( 25.00000000000000355, -5.000000000000000000, -5.750000000000000000 ) ) ;
#7421=CARTESIAN_POINT ( 'NONE',  ( 60.00000000000000000, 0.000000000000000000, -15.00000000000000355 ) ) ;
#7482=CIRCLE ( 'NONE', #991, 1.500000000000001332 ) ;
#7483=DIRECTION ( 'NONE',  ( 0.000000000000000000, 0.000000000000000000, 1.000000000000000000 ) ) ;
#7488=ADVANCED_FACE ( 'NONE', ( #4427 ), #10946, .F. ) ;
#7516=PRODUCT_DEFINITION_SHAPE ( 'NONE', 'NONE',  #10725 ) ;
#7519=LINE ( 'NONE', #9286, #5114 ) ;
#7522=CARTESIAN_POINT ( 'NONE',  ( -60.00000000000000000, -6.000000000000000000, 14.99999999999999645 ) ) ;
#7536=ORIENTED_EDGE ( 'NONE', *, *, #7722, .T. ) ;
#7543=FACE_OUTER_BOUND ( 'NONE', #3383, .T. ) ;
#7551=DIRECTION ( 'NONE',  ( -0.000000000000000000, 1.000000000000000000, -0.000000000000000000 ) ) ;
#7559=ADVANCED_FACE ( 'NONE', ( #6572 ), #9285, .F. ) ;
#7566=CARTESIAN_POINT ( 'NONE',  ( -6.666666666666660745, 0.000000000000000000, 0.000000000000000000 ) ) ;
#7587=ORIENTED_EDGE ( 'NONE', *, *, #2143, .F. ) ;
#7594=VECTOR ( 'NONE', #7986, 1000.000000000000000 ) ;
#7613=DIRECTION ( 'NONE',  ( 0.000000000000000000, 0.000000000000000000, 1.000000000000000000 ) ) ;
#7620=EDGE_LOOP ( 'NONE', ( #642, #12614, #842, #4058 ) ) ;
#7622=LINE ( 'NONE', #12666, #12276 ) ;
#7644=CARTESIAN_POINT ( 'NONE',  ( 45.00000000000000000, -5.000000000000000000, -7.250000000000000888 ) ) ;
#7647=DIRECTION ( 'NONE',  ( 0.000000000000000000, 1.000000000000000000, 0.000000000000000000 ) ) ;
#7653=CARTESIAN_POINT ( 'NONE',  ( 45.00000000000000000, 0.000000000000000000, 4.249999999999999112 ) ) ;
#7671=CONICAL_SURFACE ( 'NONE', #6207, 1.499999999999999556, 1.029744260000000189 ) ;
#7681=EDGE_CURVE ( 'NONE', #4333, #992, #3581, .T. ) ;
#7694=CARTESIAN_POINT ( 'NONE',  ( -60.00000000000000000, 0.000000000000000000, -15.00000000000000355 ) ) ;
#7696=FACE_OUTER_BOUND ( 'NONE', #8456, .T. ) ;
#7722=EDGE_CURVE ( 'NONE', #6839, #11292, #7885, .T. ) ;
#7752=CARTESIAN_POINT ( 'NONE',  ( 25.00000000000000355, -5.000000000000000000, -5.750000000000000000 ) ) ;
#7769=CARTESIAN_POINT ( 'NONE',  ( -60.00000000000000000, 0.000000000000000000, 14.99999999999999645 ) ) ;
#7789=EDGE_CURVE ( 'NONE', #376, #6806, #3021, .T. ) ;
#7834=DIRECTION ( 'NONE',  ( -0.000000000000000000, 1.000000000000000000, -0.000000000000000000 ) ) ;
#7846=VECTOR ( 'NONE', #4049, 1000.000000000000000 ) ;
#7884=CIRCLE ( 'NONE', #3726, 1.500000000000001332 ) ;
#7885=LINE ( 'NONE', #4874, #1123 ) ;
#7892=AXIS2_PLACEMENT_3D ( 'NONE', #12063, #3110, #4089 ) ;
#7893=DIRECTION ( 'NONE',  ( -0.000000000000000000, -0.000000000000000000, 1.000000000000000000 ) ) ;
#7897=CARTESIAN_POINT ( 'NONE',  ( -48.33333333333332860, 0.000000000000000000, -1.500000000000003109 ) ) ;
#7907=ORIENTED_EDGE ( 'NONE', *, *, #7722, .F. ) ;
#7911=ORIENTED_EDGE ( 'NONE', *, *, #5254, .F. ) ;
#7934=CARTESIAN_POINT ( 'NONE',  ( 25.00000000000000355, -5.000000000000000000, 5.750000000000000000 ) ) ;
#7953=FACE_OUTER_BOUND ( 'NONE', #174, .T. ) ;
#7966=EDGE_LOOP ( 'NONE', ( #3322, #8833, #7114, #6378 ) ) ;
#7971=CARTESIAN_POINT ( 'NONE',  ( -48.33333333333332860, -5.000000000000000000, 1.499999999999999556 ) ) ;
#7979=EDGE_LOOP ( 'NONE', ( #8590, #1021 ) ) ;
#7986=DIRECTION ( 'NONE',  ( -0.000000000000000000, 1.000000000000000000, -0.000000000000000000 ) ) ;
#8002=ORIENTED_EDGE ( 'NONE', *, *, #1272, .T. ) ;
#8017=CARTESIAN_POINT ( 'NONE',  ( -48.33333333333332860, -5.901290925839663970, -1.734723475976807094E-15 ) ) ;
#8034=DIRECTION ( 'NONE',  ( -0.000000000000000000, 1.000000000000000000, -0.000000000000000000 ) ) ;
#8039=DIRECTION ( 'NONE',  ( -0.000000000000000000, 1.000000000000000000, -0.000000000000000000 ) ) ;
#8048=EDGE_CURVE ( 'NONE', #39, #1413, #1131, .T. ) ;
#8061=CARTESIAN_POINT ( 'NONE',  ( 60.00000000000000000, -6.000000000000000000, 15.00000000000000000 ) ) ;
#8079=FACE_BOUND ( 'NONE', #7979, .T. ) ;
#8086=DIRECTION ( 'NONE',  ( -0.000000000000000000, 1.000000000000000000, -0.000000000000000000 ) ) ;
#8091=DIRECTION ( 'NONE',  ( -0.000000000000000000, 1.000000000000000000, -0.000000000000000000 ) ) ;
#8112=EDGE_LOOP ( 'NONE', ( #10957, #12031, #6970, #4465 ) ) ;
#8159=DIRECTION ( 'NONE',  ( -0.000000000000000000, 1.000000000000000000, -0.000000000000000000 ) ) ;
#8161=CARTESIAN_POINT ( 'NONE',  ( 25.00000000000000355, 0.000000000000000000, 5.750000000000000000 ) ) ;
#8171=CARTESIAN_POINT ( 'NONE',  ( 60.00000000000000000, -6.000000000000000000, 15.00000000000000000 ) ) ;
#8199=ADVANCED_FACE ( 'NONE', ( #5711 ), #4082, .F. ) ;
#8213=LINE ( 'NONE', #12201, #4722 ) ;
#8221=CYLINDRICAL_SURFACE ( 'NONE', #1149, 1.500000000000001332 ) ;
#8229=AXIS2_PLACEMENT_3D ( 'NONE', #3063, #7834, #12747 ) ;
#8254=CARTESIAN_POINT ( 'NONE',  ( 45.00000000000000000, -5.000000000000000000, -7.250000000000000888 ) ) ;
#8271=DIRECTION ( 'NONE',  ( -0.000000000000000000, 1.000000000000000000, -0.000000000000000000 ) ) ;
#8272=VECTOR ( 'NONE', #2922, 1000.000000000000000 ) ;
#8333=FACE_OUTER_BOUND ( 'NONE', #6079, .T. ) ;
#8336=CARTESIAN_POINT ( 'NONE',  ( -48.33333333333332860, -5.000000000000000000, -1.734723475976807094E-15 ) ) ;
#8349=ORIENTED_EDGE ( 'NONE', *, *, #2127, .F. ) ;
#8351=VERTEX_POINT ( 'NONE', #1966 ) ;
#8362=VERTEX_POINT ( 'NONE', #1836 ) ;
#8381=ORIENTED_EDGE ( 'NONE', *, *, #8598, .F. ) ;
#8387=DIRECTION ( 'NONE',  ( 1.000000000000000000, -0.000000000000000000, 0.000000000000000000 ) ) ;
#8407=STYLED_ITEM('',(#12981),#12113);
#8456=EDGE_LOOP ( 'NONE', ( #5157, #10345, #965, #6462 ) ) ;
#8480=DIRECTION ( 'NONE',  ( 0.000000000000000000, 0.000000000000000000, 1.000000000000000000 ) ) ;
#8487=CARTESIAN_POINT ( 'NONE',  ( 25.00000000000000355, -5.000000000000000000, -7.250000000000000888 ) ) ;
#8490=CARTESIAN_POINT ( 'NONE',  ( 25.00000000000000355, 0.000000000000000000, -4.249999999999998224 ) ) ;
#8499=VECTOR ( 'NONE', #8039, 1000.000000000000000 ) ;
#8522=ORIENTED_EDGE ( 'NONE', *, *, #7789, .F. ) ;
#8541=DIRECTION ( 'NONE',  ( 0.000000000000000000, 0.000000000000000000, 1.000000000000000000 ) ) ;
#8590=ORIENTED_EDGE ( 'NONE', *, *, #5202, .F. ) ;
#8598=EDGE_CURVE ( 'NONE', #309, #3927, #7519, .T. ) ;
#8633=PRODUCT_CONTEXT ( 'NONE', #2515, 'mechanical' ) ;
#8641=DIRECTION ( 'NONE',  ( -1.000000000000000000, 0.000000000000000000, -0.000000000000000000 ) ) ;
#8649=CARTESIAN_POINT ( 'NONE',  ( 45.00000000000000000, -5.000000000000000000, 4.249999999999999112 ) ) ;
#8661=CARTESIAN_POINT ( 'NONE',  ( 25.00000000000000355, -5.000000000000000000, -5.750000000000000000 ) ) ;
#8664=DIRECTION ( 'NONE',  ( 0.000000000000000000, -1.000000000000000000, 0.000000000000000000 ) ) ;
#8686=ORIENTED_EDGE ( 'NONE', *, *, #11061, .T. ) ;
#8717=( NAMED_UNIT ( * ) SI_UNIT ( $, .STERADIAN. ) SOLID_ANGLE_UNIT ( ) );
#8723=CARTESIAN_POINT ( 'NONE',  ( 45.00000000000000000, -5.000000000000000000, -4.249999999999998224 ) ) ;
#8733=AXIS2_PLACEMENT_3D ( 'NONE', #382, #8387, #10471 ) ;
#8749=CARTESIAN_POINT ( 'NONE',  ( 25.00000000000000355, 0.000000000000000000, -7.250000000000000888 ) ) ;
#8764=CONICAL_SURFACE ( 'NONE', #5632, 1.500000000000001332, 1.029744260000000633 ) ;
#8798=ORIENTED_EDGE ( 'NONE', *, *, #4286, .F. ) ;
#8833=ORIENTED_EDGE ( 'NONE', *, *, #5921, .F. ) ;
#8838=DIRECTION ( 'NONE',  ( -0.000000000000000000, 1.000000000000000000, -0.000000000000000000 ) ) ;
#8861=AXIS2_PLACEMENT_3D ( 'NONE', #2522, #469, #9513 ) ;
#8865=EDGE_CURVE ( 'NONE', #11250, #4553, #3790, .T. ) ;
#8874=( NAMED_UNIT ( * ) PLANE_ANGLE_UNIT ( ) SI_UNIT ( $, .RADIAN. ) );
#8883=DIRECTION ( 'NONE',  ( 0.000000000000000000, 0.000000000000000000, 1.000000000000000000 ) ) ;
#8912=DIRECTION ( 'NONE',  ( -0.000000000000000000, 1.000000000000000000, -0.000000000000000000 ) ) ;
#8933=LINE ( 'NONE', #3782, #12267 ) ;
#8945=CARTESIAN_POINT ( 'NONE',  ( 45.00000000000000000, -5.000000000000000000, 5.750000000000000888 ) ) ;
#8989=FACE_OUTER_BOUND ( 'NONE', #4632, .T. ) ;
#8990=CONICAL_SURFACE ( 'NONE', #1904, 1.500000000000001332, 1.029744260000000411 ) ;
#8995=ORIENTED_EDGE ( 'NONE', *, *, #1200, .T. ) ;
#8997=CARTESIAN_POINT ( 'NONE',  ( 0.000000000000000000, 0.000000000000000000, 0.000000000000000000 ) ) ;
#9004=DIRECTION ( 'NONE',  ( -0.000000000000000000, 1.000000000000000000, -0.000000000000000000 ) ) ;
#9008=AXIS2_PLACEMENT_3D ( 'NONE', #964, #2463, #12090 ) ;
#9039=ADVANCED_FACE ( 'NONE', ( #3570 ), #11075, .F. ) ;
#9058=ORIENTED_EDGE ( 'NONE', *, *, #4742, .T. ) ;
#9098=CARTESIAN_POINT ( 'NONE',  ( 45.00000000000000000, -5.000000000000000000, 5.750000000000000888 ) ) ;
#9109=CARTESIAN_POINT ( 'NONE',  ( -60.00000000000000000, -6.000000000000000000, -15.00000000000000355 ) ) ;
#9128=CIRCLE ( 'NONE', #3506, 1.500000000000001332 ) ;
#9130=CARTESIAN_POINT ( 'NONE',  ( 45.00000000000000000, 0.000000000000000000, 5.750000000000000888 ) ) ;
#9135=CARTESIAN_POINT ( 'NONE',  ( -6.666666666666660745, 0.000000000000000000, 0.000000000000000000 ) ) ;
#9148=ORIENTED_EDGE ( 'NONE', *, *, #7681, .T. ) ;
#9180=EDGE_CURVE ( 'NONE', #12248, #1413, #6690, .T. ) ;
#9213=ORIENTED_EDGE ( 'NONE', *, *, #3328, .T. ) ;
#9272=AXIS2_PLACEMENT_3D ( 'NONE', #8161, #7243, #2142 ) ;
#9274=ORIENTED_EDGE ( 'NONE', *, *, #4723, .F. ) ;
#9278=DIRECTION ( 'NONE',  ( -2.891205793294678696E-17, 0.000000000000000000, 1.000000000000000000 ) ) ;
#9280=EDGE_CURVE ( 'NONE', #6649, #309, #9600, .T. ) ;
#9285=CONICAL_SURFACE ( 'NONE', #3860, 1.500000000000001332, 1.029744260000000633 ) ;
#9286=CARTESIAN_POINT ( 'NONE',  ( -6.666666666666660745, 0.000000000000000000, 1.499999999999999556 ) ) ;
#9303=DIRECTION ( 'NONE',  ( -1.000000000000000000, -0.000000000000000000, -0.000000000000000000 ) ) ;
#9331=DIRECTION ( 'NONE',  ( -0.000000000000000000, 1.000000000000000000, -0.000000000000000000 ) ) ;
#9333=ORIENTED_EDGE ( 'NONE', *, *, #5118, .F. ) ;
#9336=ORIENTED_EDGE ( 'NONE', *, *, #2250, .T. ) ;
#9349=EDGE_LOOP ( 'NONE', ( #11919, #10978, #10934 ) ) ;
#9439=CARTESIAN_POINT ( 'NONE',  ( 60.00000000000000000, -6.000000000000000000, -15.00000000000000355 ) ) ;
#9441=CARTESIAN_POINT ( 'NONE',  ( -6.666666666666660745, -5.000000000000000000, -1.499999999999999556 ) ) ;
#9450=ORIENTED_EDGE ( 'NONE', *, *, #3048, .F. ) ;
#9460=EDGE_CURVE ( 'NONE', #6459, #6839, #1314, .T. ) ;
#9486=ORIENTED_EDGE ( 'NONE', *, *, #2143, .T. ) ;
#9488=PLANE ( 'NONE',  #8733 ) ;
#9506=DIRECTION ( 'NONE',  ( 0.000000000000000000, 0.000000000000000000, 1.000000000000000000 ) ) ;
#9513=DIRECTION ( 'NONE',  ( 0.000000000000000000, 0.000000000000000000, 1.000000000000000000 ) ) ;
#9521=CIRCLE ( 'NONE', #1162, 1.500000000000001332 ) ;
#9549=PLANE ( 'NONE',  #12005 ) ;
#9551=VECTOR ( 'NONE', #4135, 1000.000000000000000 ) ;
#9572=CARTESIAN_POINT ( 'NONE',  ( 25.00000000000000355, 0.000000000000000000, -5.750000000000000000 ) ) ;
#9589=DIRECTION ( 'NONE',  ( -0.000000000000000000, 1.000000000000000000, -0.000000000000000000 ) ) ;
#9600=CIRCLE ( 'NONE', #7301, 1.499999999999999556 ) ;
#9602=VERTEX_POINT ( 'NONE', #8649 ) ;
#9634=DIRECTION ( 'NONE',  ( 0.000000000000000000, 0.000000000000000000, 1.000000000000000000 ) ) ;
#9636=AXIS2_PLACEMENT_3D ( 'NONE', #511, #6667, #646 ) ;
#9645=FACE_OUTER_BOUND ( 'NONE', #9852, .T. ) ;
#9730=CONICAL_SURFACE ( 'NONE', #1379, 1.500000000000001332, 1.029744260000000411 ) ;
#9746=EDGE_CURVE ( 'NONE', #376, #7167, #7000, .T. ) ;
#9797=FACE_OUTER_BOUND ( 'NONE', #4970, .T. ) ;
#9800=CYLINDRICAL_SURFACE ( 'NONE', #10962, 1.499999999999999556 ) ;
#9852=EDGE_LOOP ( 'NONE', ( #968, #3464, #9877 ) ) ;
#9858=LINE ( 'NONE', #886, #11361 ) ;
#9863=EDGE_LOOP ( 'NONE', ( #1234, #9450, #1150, #11321 ) ) ;
#9871=CONICAL_SURFACE ( 'NONE', #5059, 1.500000000000001332, 1.029744260000000411 ) ;
#9877=ORIENTED_EDGE ( 'NONE', *, *, #3048, .T. ) ;
#9887=DIRECTION ( 'NONE',  ( 0.000000000000000000, 0.000000000000000000, 1.000000000000000000 ) ) ;
#9907=CLOSED_SHELL ( 'NONE', ( #6918, #10626, #4390, #11722, #3362, #1943, #8199, #11883, #11261, #1850, #9039, #10149, #5513, #5992, #1322, #12473, #2201, #6240, #141, #5296, #3041, #10794, #223, #6559, #10272, #12827, #1458, #7488, #873, #7559 ) ) ;
#9916=ORIENTED_EDGE ( 'NONE', *, *, #7789, .T. ) ;
#9938=DIRECTION ( 'NONE',  ( -0.000000000000000000, 1.000000000000000000, -0.000000000000000000 ) ) ;
#9942=ORIENTED_EDGE ( 'NONE', *, *, #1200, .F. ) ;
#9950=CARTESIAN_POINT ( 'NONE',  ( 60.00000000000000000, 0.000000000000000000, 15.00000000000000000 ) ) ;
#9973=CARTESIAN_POINT ( 'NONE',  ( 45.00000000000000000, 0.000000000000000000, -5.750000000000000000 ) ) ;
#9982=EDGE_CURVE ( 'NONE', #7180, #3927, #1461, .T. ) ;
#9993=VERTEX_POINT ( 'NONE', #7175 ) ;
#9995=FACE_OUTER_BOUND ( 'NONE', #9349, .T. ) ;
#10039=DIRECTION ( 'NONE',  ( 0.000000000000000000, 0.000000000000000000, 1.000000000000000000 ) ) ;
#10043=EDGE_LOOP ( 'NONE', ( #8522, #7236, #2809, #11716 ) ) ;
#10049=DIRECTION ( 'NONE',  ( 1.000000000000000000, 0.000000000000000000, 2.891205793294678696E-17 ) ) ;
#10061=ORIENTED_EDGE ( 'NONE', *, *, #8865, .T. ) ;
#10109=EDGE_CURVE ( 'NONE', #12765, #6375, #827, .T. ) ;
#10121=CARTESIAN_POINT ( 'NONE',  ( -48.33333333333332860, 0.000000000000000000, -1.734723475976807094E-15 ) ) ;
#10125=VECTOR ( 'NONE', #7647, 1000.000000000000000 ) ;
#10145=AXIS2_PLACEMENT_3D ( 'NONE', #10431, #6627, #4417 ) ;
#10149=ADVANCED_FACE ( 'NONE', ( #2600 ), #6320, .F. ) ;
#10154=EDGE_LOOP ( 'NONE', ( #3481, #1429, #9916 ) ) ;
#10160=ORIENTED_EDGE ( 'NONE', *, *, #4286, .T. ) ;
#10173=VERTEX_POINT ( 'NONE', #7371 ) ;
#10182=ORIENTED_EDGE ( 'NONE', *, *, #2697, .F. ) ;
#10272=ADVANCED_FACE ( 'NONE', ( #7696 ), #6708, .F. ) ;
#10283=ORIENTED_EDGE ( 'NONE', *, *, #10948, .T. ) ;
#10303=DIRECTION ( 'NONE',  ( 0.000000000000000000, 0.000000000000000000, 1.000000000000000000 ) ) ;
#10308=DIRECTION ( 'NONE',  ( 0.000000000000000000, 0.000000000000000000, 1.000000000000000000 ) ) ;
#10340=CARTESIAN_POINT ( 'NONE',  ( 25.00000000000000355, -5.901290925839664858, -5.750000000000000000 ) ) ;
#10345=ORIENTED_EDGE ( 'NONE', *, *, #2250, .F. ) ;
#10350=CARTESIAN_POINT ( 'NONE',  ( -60.00000000000000000, -6.000000000000000000, -15.00000000000000355 ) ) ;
#10396=ORIENTED_EDGE ( 'NONE', *, *, #5870, .T. ) ;
#10414=VECTOR ( 'NONE', #8091, 1000.000000000000000 ) ;
#10422=LINE ( 'NONE', #11530, #12504 ) ;
#10431=CARTESIAN_POINT ( 'NONE',  ( 45.00000000000000000, -5.000000000000000000, 5.750000000000000888 ) ) ;
#10436=DIRECTION ( 'NONE',  ( -0.000000000000000000, 1.000000000000000000, -0.000000000000000000 ) ) ;
#10462=DIRECTION ( 'NONE',  ( 0.000000000000000000, 0.000000000000000000, 1.000000000000000000 ) ) ;
#10471=DIRECTION ( 'NONE',  ( 0.000000000000000000, 0.000000000000000000, -1.000000000000000000 ) ) ;
#10535=FACE_OUTER_BOUND ( 'NONE', #11041, .T. ) ;
#10551=AXIS2_PLACEMENT_3D ( 'NONE', #12458, #1660, #7483 ) ;
#10565=CARTESIAN_POINT ( 'NONE',  ( -48.33333333333332860, -5.000000000000000000, -1.734723475976807094E-15 ) ) ;
#10585=CARTESIAN_POINT ( 'NONE',  ( -6.666666666666660745, -5.000000000000000000, 0.000000000000000000 ) ) ;
#10626=ADVANCED_FACE ( 'NONE', ( #3316 ), #11410, .F. ) ;
#10644=DIRECTION ( 'NONE',  ( -0.000000000000000000, 1.000000000000000000, -0.000000000000000000 ) ) ;
#10650=AXIS2_PLACEMENT_3D ( 'NONE', #9135, #226, #11950 ) ;
#10653=CARTESIAN_POINT ( 'NONE',  ( -60.00000000000000000, -6.000000000000000000, 14.99999999999999645 ) ) ;
#10660=ORIENTED_EDGE ( 'NONE', *, *, #12311, .T. ) ;
#10662=FACE_OUTER_BOUND ( 'NONE', #5201, .T. ) ;
#10698=LINE ( 'NONE', #7694, #5948 ) ;
#10722=ORIENTED_EDGE ( 'NONE', *, *, #5921, .T. ) ;
#10725=PRODUCT_DEFINITION ( 'UNKNOWN', '', #1762, #4215 ) ;
#10753=ORIENTED_EDGE ( 'NONE', *, *, #168, .F. ) ;
#10765=DIRECTION ( 'NONE',  ( -0.000000000000000000, 1.000000000000000000, -0.000000000000000000 ) ) ;
#10773=FILL_AREA_STYLE ('',( #10895 ) ) ;
#10774=FACE_BOUND ( 'NONE', #4959, .T. ) ;
#10780=CARTESIAN_POINT ( 'NONE',  ( 45.00000000000000000, -5.000000000000000000, 4.249999999999999112 ) ) ;
#10783=LINE ( 'NONE', #7522, #10125 ) ;
#10794=ADVANCED_FACE ( 'NONE', ( #9645 ), #4206, .F. ) ;
#10811=CARTESIAN_POINT ( 'NONE',  ( -6.666666666666660745, -5.000000000000000000, 0.000000000000000000 ) ) ;
#10815=ORIENTED_EDGE ( 'NONE', *, *, #5141, .T. ) ;
#10825=DIRECTION ( 'NONE',  ( 0.000000000000000000, 0.000000000000000000, 1.000000000000000000 ) ) ;
#10837=LINE ( 'NONE', #7897, #10414 ) ;
#10839=CYLINDRICAL_SURFACE ( 'NONE', #8229, 1.500000000000001332 ) ;
#10846=LINE ( 'NONE', #7971, #7846 ) ;
#10857=VERTEX_POINT ( 'NONE', #11540 ) ;
#10867=DIRECTION ( 'NONE',  ( -0.000000000000000000, 1.000000000000000000, -0.000000000000000000 ) ) ;
#10895=FILL_AREA_STYLE_COLOUR ( '', #40 ) ;
#10908=FACE_OUTER_BOUND ( 'NONE', #12696, .T. ) ;
#10934=ORIENTED_EDGE ( 'NONE', *, *, #5436, .T. ) ;
#10946=CONICAL_SURFACE ( 'NONE', #714, 1.499999999999999556, 1.029744260000000189 ) ;
#10948=EDGE_CURVE ( 'NONE', #6839, #10173, #1990, .T. ) ;
#10957=ORIENTED_EDGE ( 'NONE', *, *, #4353, .F. ) ;
#10962=AXIS2_PLACEMENT_3D ( 'NONE', #4894, #8034, #8883 ) ;
#10963=LINE ( 'NONE', #10780, #11986 ) ;
#10971=AXIS2_PLACEMENT_3D ( 'NONE', #9973, #10765, #5980 ) ;
#10978=ORIENTED_EDGE ( 'NONE', *, *, #168, .T. ) ;
#11015=DIRECTION ( 'NONE',  ( -0.000000000000000000, 1.000000000000000000, -0.000000000000000000 ) ) ;
#11021=EDGE_LOOP ( 'NONE', ( #10753, #5029, #9336 ) ) ;
#11024=CARTESIAN_POINT ( 'NONE',  ( 45.00000000000000000, 0.000000000000000000, -5.750000000000000000 ) ) ;
#11041=EDGE_LOOP ( 'NONE', ( #3088, #5722, #5498, #8381 ) ) ;
#11042=VECTOR ( 'NONE', #12623, 1000.000000000000000 ) ;
#11050=ORIENTED_EDGE ( 'NONE', *, *, #10109, .T. ) ;
#11058=ORIENTED_EDGE ( 'NONE', *, *, #1544, .F. ) ;
#11061=EDGE_CURVE ( 'NONE', #39, #11476, #3897, .T. ) ;
#11075=CONICAL_SURFACE ( 'NONE', #5438, 1.500000000000001332, 1.029744260000000411 ) ;
#11085=LINE ( 'NONE', #5068, #6830 ) ;
#11093=CARTESIAN_POINT ( 'NONE',  ( 45.00000000000000000, 0.000000000000000000, 5.750000000000000888 ) ) ;
#11141=VECTOR ( 'NONE', #3710, 999.9999999999998863 ) ;
#11156=DIRECTION ( 'NONE',  ( 0.000000000000000000, 0.000000000000000000, 1.000000000000000000 ) ) ;
#11173=AXIS2_PLACEMENT_3D ( 'NONE', #11093, #4306, #11227 ) ;
#11210=DIRECTION ( 'NONE',  ( 0.000000000000000000, -1.000000000000000000, 0.000000000000000000 ) ) ;
#11227=DIRECTION ( 'NONE',  ( 0.000000000000000000, 0.000000000000000000, 1.000000000000000000 ) ) ;
#11230=CONICAL_SURFACE ( 'NONE', #3934, 1.500000000000001332, 1.029744260000000411 ) ;
#11242=ORIENTED_EDGE ( 'NONE', *, *, #4742, .F. ) ;
#11250=VERTEX_POINT ( 'NONE', #12257 ) ;
#11261=ADVANCED_FACE ( 'NONE', ( #8333 ), #8990, .F. ) ;
#11262=VERTEX_POINT ( 'NONE', #7345 ) ;
#11285=CARTESIAN_POINT ( 'NONE',  ( -48.33333333333332860, 0.000000000000000000, -1.734723475976807094E-15 ) ) ;
#11287=CARTESIAN_POINT ( 'NONE',  ( -6.666666666666660745, -5.000000000000000000, 0.000000000000000000 ) ) ;
#11292=VERTEX_POINT ( 'NONE', #11595 ) ;
#11301=CARTESIAN_POINT ( 'NONE',  ( -6.666666666666660745, -5.000000000000000000, 0.000000000000000000 ) ) ;
#11306=DIRECTION ( 'NONE',  ( -0.000000000000000000, 1.000000000000000000, -0.000000000000000000 ) ) ;
#11321=ORIENTED_EDGE ( 'NONE', *, *, #5202, .T. ) ;
#11336=AXIS2_PLACEMENT_3D ( 'NONE', #12697, #3546, #8641 ) ;
#11344=ORIENTED_EDGE ( 'NONE', *, *, #1861, .T. ) ;
#11356=ADVANCED_BREP_SHAPE_REPRESENTATION ( '', ( #12113, #5704 ), #3631 ) ;
#11361=VECTOR ( 'NONE', #10049, 1000.000000000000000 ) ;
#11410=CYLINDRICAL_SURFACE ( 'NONE', #2528, 1.500000000000001332 ) ;
#11427=CIRCLE ( 'NONE', #4545, 1.500000000000001332 ) ;
#11450=UNCERTAINTY_MEASURE_WITH_UNIT (LENGTH_MEASURE( 1.000000000000000082E-05 ), #11723, 'distance_accuracy_value', 'NONE');
#11476=VERTEX_POINT ( 'NONE', #3018 ) ;
#11480=PRODUCT ( 'base plate', 'base plate', '', ( #8633 ) ) ;
#11489=DIRECTION ( 'NONE',  ( 0.000000000000000000, 0.000000000000000000, 1.000000000000000000 ) ) ;
#11530=CARTESIAN_POINT ( 'NONE',  ( 60.00000000000000000, -6.000000000000000000, -15.00000000000000355 ) ) ;
#11531=EDGE_CURVE ( 'NONE', #2096, #4006, #5830, .T. ) ;
#11540=CARTESIAN_POINT ( 'NONE',  ( 25.00000000000000355, -5.000000000000000000, 7.250000000000000888 ) ) ;
#11578=CYLINDRICAL_SURFACE ( 'NONE', #9636, 1.499999999999999556 ) ;
#11595=CARTESIAN_POINT ( 'NONE',  ( -60.00000000000000000, -6.000000000000000000, 14.99999999999999645 ) ) ;
#11653=VERTEX_POINT ( 'NONE', #10340 ) ;
#11702=EDGE_LOOP ( 'NONE', ( #2825, #2376 ) ) ;
#11713=EDGE_LOOP ( 'NONE', ( #3171, #6953, #7536, #8995 ) ) ;
#11716=ORIENTED_EDGE ( 'NONE', *, *, #1861, .F. ) ;
#11722=ADVANCED_FACE ( 'NONE', ( #10535 ), #11578, .F. ) ;
#11723=( LENGTH_UNIT ( ) NAMED_UNIT ( * ) SI_UNIT ( .MILLI., .METRE. ) );
#11726=CARTESIAN_POINT ( 'NONE',  ( -60.00000000000000000, -6.000000000000000000, -15.00000000000000355 ) ) ;
#11732=DIRECTION ( 'NONE',  ( 0.000000000000000000, 0.000000000000000000, 1.000000000000000000 ) ) ;
#11740=VECTOR ( 'NONE', #248, 999.9999999999998863 ) ;
#11813=CIRCLE ( 'NONE', #11173, 1.500000000000001332 ) ;
#11827=DIRECTION ( 'NONE',  ( 1.049727191973305517E-16, 0.5150380737757253025, -0.8571673013836857979 ) ) ;
#11883=ADVANCED_FACE ( 'NONE', ( #10908 ), #836, .F. ) ;
#11904=ORIENTED_EDGE ( 'NONE', *, *, #2299, .T. ) ;
#11915=CARTESIAN_POINT ( 'NONE',  ( 45.00000000000000000, -5.901290925839664858, -5.750000000000000000 ) ) ;
#11919=ORIENTED_EDGE ( 'NONE', *, *, #5954, .F. ) ;
#11920=AXIS2_PLACEMENT_3D ( 'NONE', #12594, #2585, #11732 ) ;
#11921=DIRECTION ( 'NONE',  ( 0.000000000000000000, 0.000000000000000000, 1.000000000000000000 ) ) ;
#11928=DIRECTION ( 'NONE',  ( -0.000000000000000000, 1.000000000000000000, -0.000000000000000000 ) ) ;
#11948=ORIENTED_EDGE ( 'NONE', *, *, #4918, .F. ) ;
#11950=DIRECTION ( 'NONE',  ( 0.000000000000000000, 0.000000000000000000, 1.000000000000000000 ) ) ;
#11959=ORIENTED_EDGE ( 'NONE', *, *, #57, .F. ) ;
#11969=EDGE_CURVE ( 'NONE', #992, #1427, #1500, .T. ) ;
#11986=VECTOR ( 'NONE', #11827, 999.9999999999998863 ) ;
#12005=AXIS2_PLACEMENT_3D ( 'NONE', #10653, #572, #4579 ) ;
#12026=CIRCLE ( 'NONE', #3263, 1.500000000000001332 ) ;
#12031=ORIENTED_EDGE ( 'NONE', *, *, #12704, .F. ) ;
#12040=CARTESIAN_POINT ( 'NONE',  ( 25.00000000000000355, 0.000000000000000000, 4.249999999999998224 ) ) ;
#12063=CARTESIAN_POINT ( 'NONE',  ( 25.00000000000000355, -5.000000000000000000, -5.750000000000000000 ) ) ;
#12090=DIRECTION ( 'NONE',  ( 0.000000000000000000, 0.000000000000000000, 1.000000000000000000 ) ) ;
#12104=FACE_OUTER_BOUND ( 'NONE', #6866, .T. ) ;
#12113=MANIFOLD_SOLID_BREP ( 'AdvancedHole2', #9907 ) ;
#12123=EDGE_LOOP ( 'NONE', ( #2167, #2658, #3229, #10061 ) ) ;
#12147=DIRECTION ( 'NONE',  ( -0.000000000000000000, 1.000000000000000000, -0.000000000000000000 ) ) ;
#12192=DIRECTION ( 'NONE',  ( -0.000000000000000000, 1.000000000000000000, -0.000000000000000000 ) ) ;
#12201=CARTESIAN_POINT ( 'NONE',  ( -6.666666666666660745, -5.000000000000000000, 1.499999999999999556 ) ) ;
#12203=DIRECTION ( 'NONE',  ( -0.000000000000000000, 1.000000000000000000, -0.000000000000000000 ) ) ;
#12204=DIRECTION ( 'NONE',  ( 0.000000000000000000, 0.000000000000000000, 1.000000000000000000 ) ) ;
#12248=VERTEX_POINT ( 'NONE', #11915 ) ;
#12257=CARTESIAN_POINT ( 'NONE',  ( -60.00000000000000000, 0.000000000000000000, 14.99999999999999645 ) ) ;
#12261=CARTESIAN_POINT ( 'NONE',  ( 25.00000000000000355, -5.000000000000000000, -7.250000000000000888 ) ) ;
#12267=VECTOR ( 'NONE', #7893, 1000.000000000000000 ) ;
#12271=CARTESIAN_POINT ( 'NONE',  ( 25.00000000000000355, 0.000000000000000000, -5.750000000000000000 ) ) ;
#12276=VECTOR ( 'NONE', #10436, 1000.000000000000000 ) ;
#12277=SHAPE_REPRESENTATION_RELATIONSHIP ( 'NONE' , 'NONE' ,  #5503, #11356 ) ;
#12311=EDGE_CURVE ( 'NONE', #12248, #39, #2307, .T. ) ;
#12320=CARTESIAN_POINT ( 'NONE',  ( 45.00000000000000000, -5.000000000000000000, -5.750000000000000000 ) ) ;
#12325=FACE_OUTER_BOUND ( 'NONE', #12123, .T. ) ;
#12341=DIRECTION ( 'NONE',  ( -0.000000000000000000, 1.000000000000000000, -0.000000000000000000 ) ) ;
#12355=CARTESIAN_POINT ( 'NONE',  ( -60.00000000000000000, -6.000000000000000000, 14.99999999999999645 ) ) ;
#12358=ORIENTED_EDGE ( 'NONE', *, *, #9746, .F. ) ;
#12391=DIRECTION ( 'NONE',  ( -0.000000000000000000, 1.000000000000000000, -0.000000000000000000 ) ) ;
#12418=EDGE_CURVE ( 'NONE', #2970, #10857, #3739, .T. ) ;
#12447=LINE ( 'NONE', #4532, #4257 ) ;
#12454=AXIS2_PLACEMENT_3D ( 'NONE', #6045, #11015, #10039 ) ;
#12458=CARTESIAN_POINT ( 'NONE',  ( 45.00000000000000000, -5.000000000000000000, -5.750000000000000000 ) ) ;
#12473=ADVANCED_FACE ( 'NONE', ( #10662 ), #4653, .T. ) ;
#12488=DIRECTION ( 'NONE',  ( 1.000000000000000000, 0.000000000000000000, 2.891205793294678696E-17 ) ) ;
#12504=VECTOR ( 'NONE', #12519, 1000.000000000000000 ) ;
#12515=ORIENTED_EDGE ( 'NONE', *, *, #3328, .F. ) ;
#12519=DIRECTION ( 'NONE',  ( 0.000000000000000000, 1.000000000000000000, 0.000000000000000000 ) ) ;
#12552=ORIENTED_EDGE ( 'NONE', *, *, #3804, .T. ) ;
#12594=CARTESIAN_POINT ( 'NONE',  ( 45.00000000000000000, -5.000000000000000000, -5.750000000000000000 ) ) ;
#12614=ORIENTED_EDGE ( 'NONE', *, *, #7283, .T. ) ;
#12623=DIRECTION ( 'NONE',  ( 1.000000000000000000, 0.000000000000000000, 2.891205793294678696E-17 ) ) ;
#12637=UNCERTAINTY_MEASURE_WITH_UNIT (LENGTH_MEASURE( 1.000000000000000082E-05 ), #2073, 'distance_accuracy_value', 'NONE');
#12645=VECTOR ( 'NONE', #4708, 1000.000000000000000 ) ;
#12666=CARTESIAN_POINT ( 'NONE',  ( 25.00000000000000355, 0.000000000000000000, 7.250000000000000888 ) ) ;
#12668=CARTESIAN_POINT ( 'NONE',  ( -48.33333333333332860, -5.000000000000000000, -1.734723475976807094E-15 ) ) ;
#12678=FACE_OUTER_BOUND ( 'NONE', #5329, .T. ) ;
#12696=EDGE_LOOP ( 'NONE', ( #8798, #6968, #11050, #11948 ) ) ;
#12697=CARTESIAN_POINT ( 'NONE',  ( -60.00000000000000000, -6.000000000000000000, -15.00000000000000355 ) ) ;
#12704=EDGE_CURVE ( 'NONE', #8351, #4553, #4249, .T. ) ;
#12717=DIRECTION ( 'NONE',  ( -0.000000000000000000, 1.000000000000000000, -0.000000000000000000 ) ) ;
#12747=DIRECTION ( 'NONE',  ( 0.000000000000000000, 0.000000000000000000, 1.000000000000000000 ) ) ;
#12757=CARTESIAN_POINT ( 'NONE',  ( 25.00000000000000355, -5.000000000000000000, 7.250000000000000888 ) ) ;
#12765=VERTEX_POINT ( 'NONE', #691 ) ;
#12793=CYLINDRICAL_SURFACE ( 'NONE', #12454, 1.500000000000001332 ) ;
#12827=ADVANCED_FACE ( 'NONE', ( #2740 ), #9871, .F. ) ;
#12838=CARTESIAN_POINT ( 'NONE',  ( -48.33333333333332860, -5.000000000000000000, -1.734723475976807094E-15 ) ) ;
#12859=CIRCLE ( 'NONE', #1580, 1.500000000000001332 ) ;
#12907=DIRECTION ( 'NONE',  ( 0.000000000000000000, 0.000000000000000000, 1.000000000000000000 ) ) ;
#12975=COLOUR_RGB('Dark Blue',0.08,0.2,0.34);
#12976=FILL_AREA_STYLE_COLOUR('',#12975);
#12977=FILL_AREA_STYLE('',(#12976));
#12978=SURFACE_STYLE_FILL_AREA(#12977);
#12979=SURFACE_SIDE_STYLE('',(#12978));
#12980=SURFACE_STYLE_USAGE(.BOTH.,#12979);
#12981=PRESENTATION_STYLE_ASSIGNMENT((#12980));
ENDSEC;
END-ISO-10303-21;
